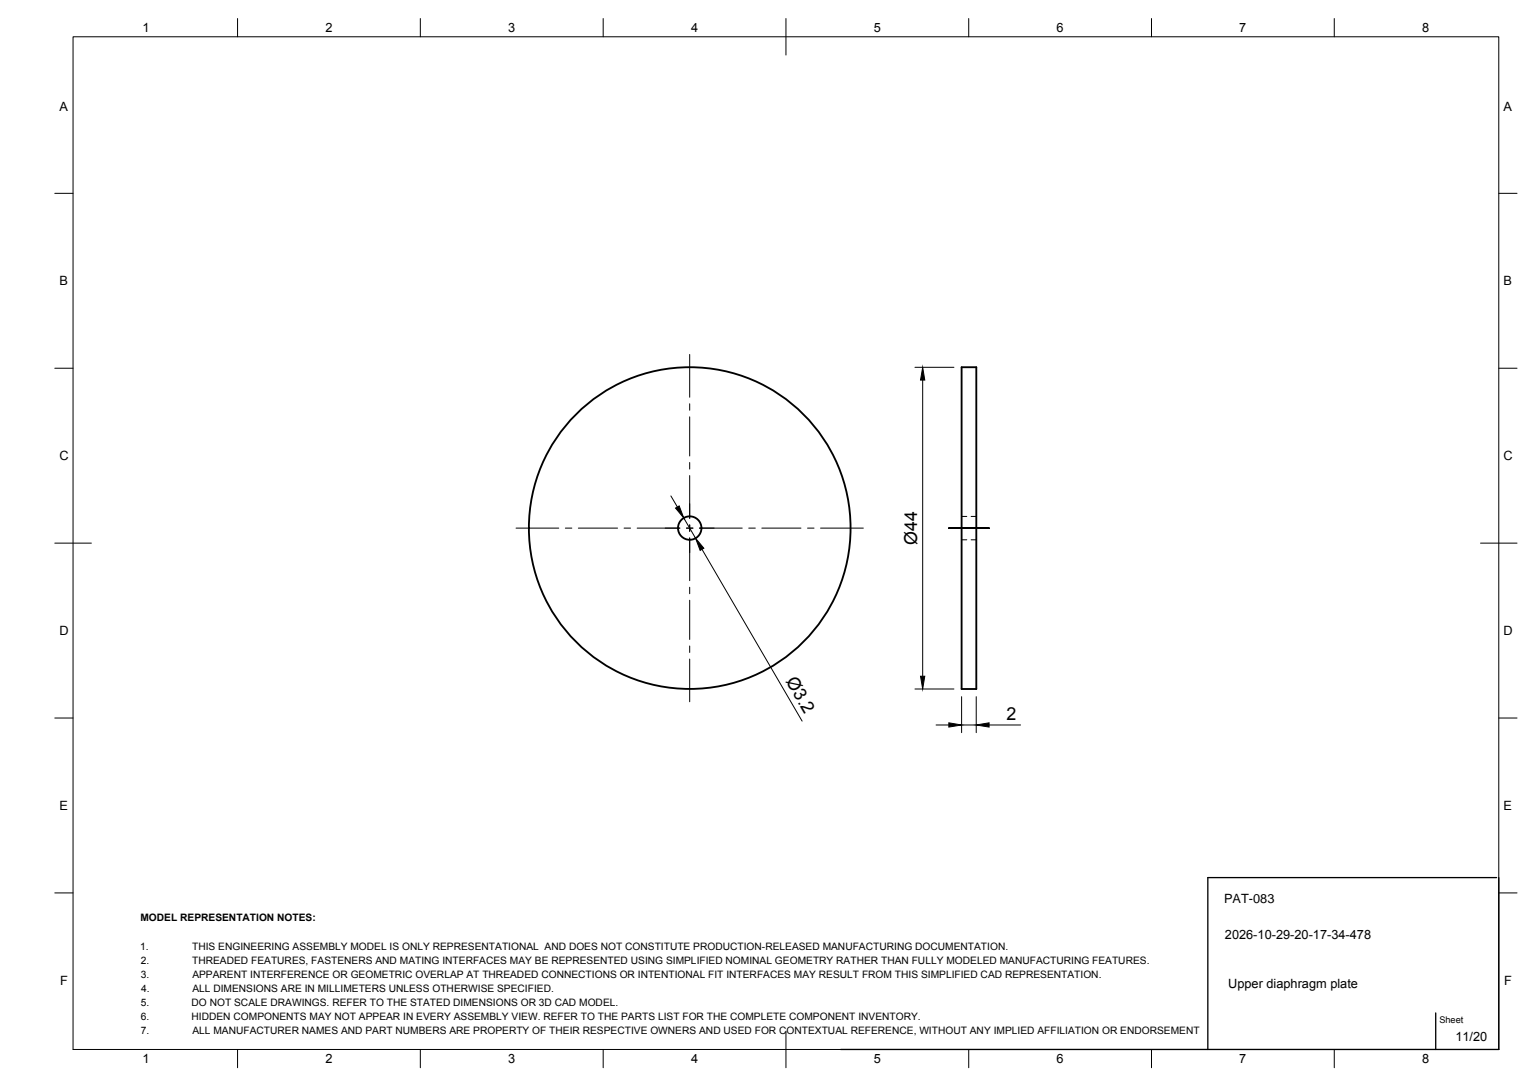
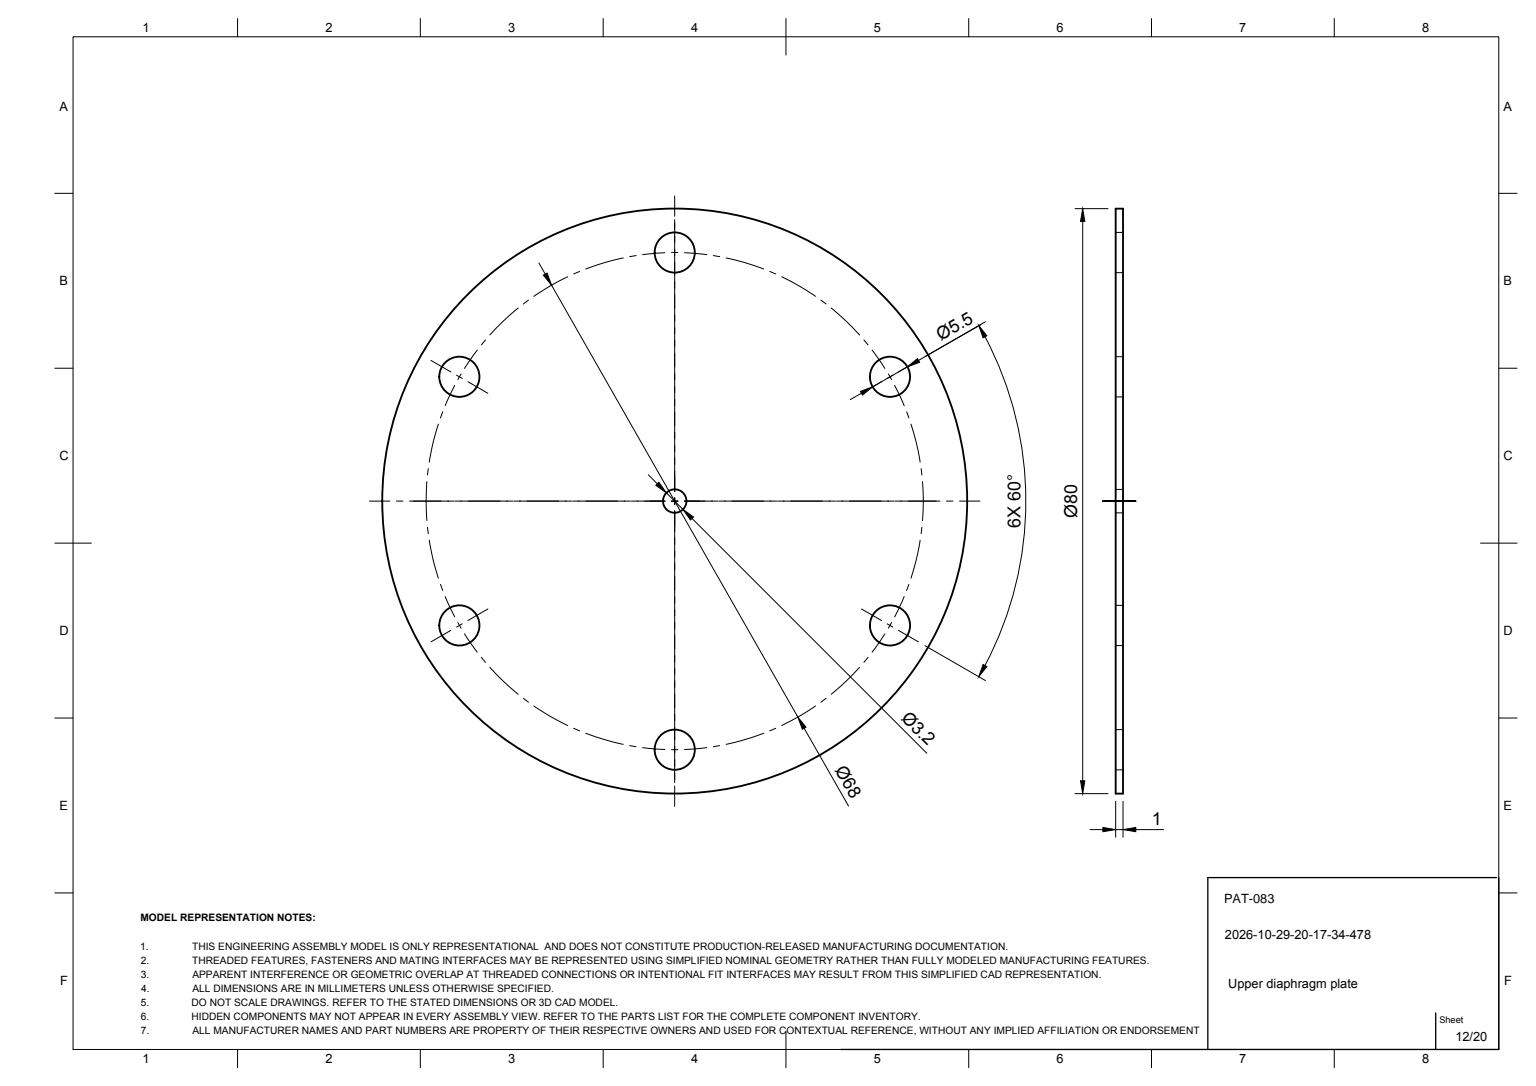
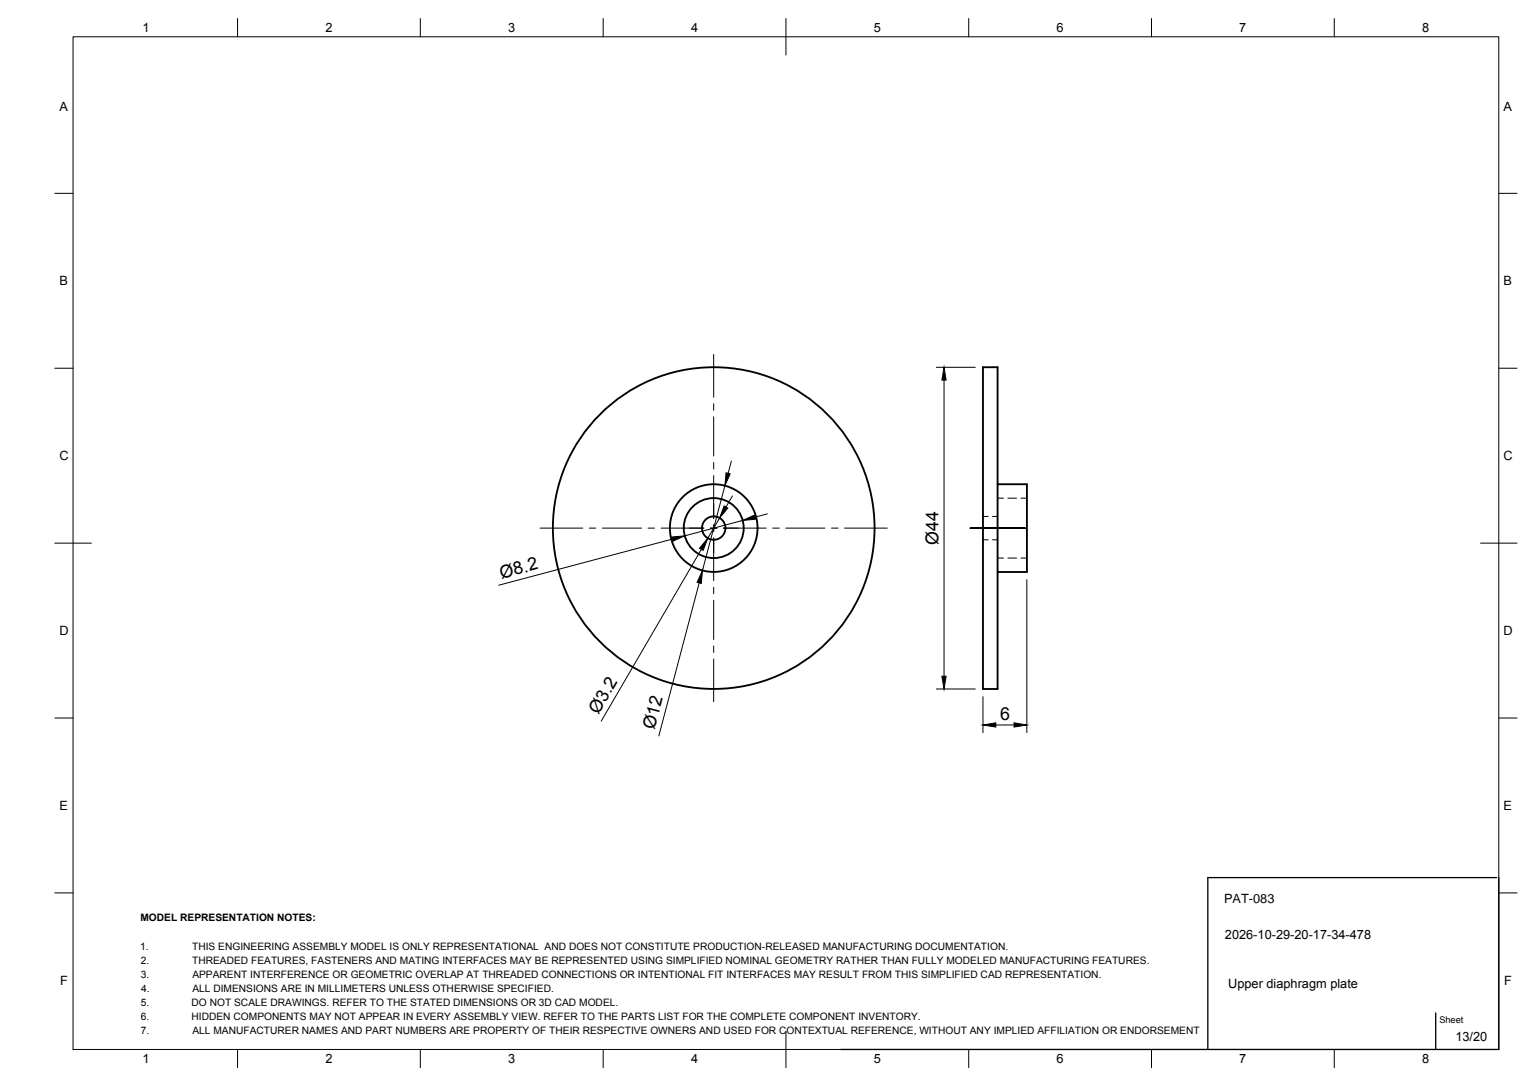
ISO-10303-21;
HEADER;
/* Generated by software containing ST-Developer
 * from STEP Tools, Inc. (www.steptools.com) 
 */

FILE_DESCRIPTION(
/* description */ ('PAT-083'),
/* implementation_level */ '2;1');

FILE_NAME(
/* name */ 'Upper diaphragm plate.step',
/* time_stamp */ '2026-10-29T20:18:00-07:00',
/* author */ (''),
/* organization */ (''),
/* preprocessor_version */ 'ST-DEVELOPER v20.2',
/* originating_system */ 'Autodesk Translation Framework v15.17.0.0',
/* authorisation */ '');

FILE_SCHEMA (('AUTOMOTIVE_DESIGN { 1 0 10303 214 3 1 1 }'));
ENDSEC;

DATA;
#10=MECHANICAL_DESIGN_GEOMETRIC_PRESENTATION_REPRESENTATION('',(#239),#8428);
#191=SHAPE_REPRESENTATION_RELATIONSHIP('SRR','None',#8525,#215);
#215=ADVANCED_BREP_SHAPE_REPRESENTATION('',(#263),#8414);
#239=STYLED_ITEM('',(#8698),#263);
#263=MANIFOLD_SOLID_BREP('Body1',#3685);
#320=FACE_BOUND('',#869,.T.);
#321=FACE_BOUND('',#871,.T.);
#322=FACE_BOUND('',#875,.T.);
#323=FACE_BOUND('',#877,.T.);
#407=PLANE('',#4156);
#408=PLANE('',#4157);
#409=PLANE('',#4164);
#410=PLANE('',#4165);
#588=FACE_OUTER_BOUND('',#866,.T.);
#589=FACE_OUTER_BOUND('',#867,.T.);
#590=FACE_OUTER_BOUND('',#868,.T.);
#591=FACE_OUTER_BOUND('',#870,.T.);
#592=FACE_OUTER_BOUND('',#872,.T.);
#593=FACE_OUTER_BOUND('',#873,.T.);
#594=FACE_OUTER_BOUND('',#874,.T.);
#595=FACE_OUTER_BOUND('',#876,.T.);
#866=EDGE_LOOP('',(#2804,#2805,#2806,#2807));
#867=EDGE_LOOP('',(#2808,#2809,#2810,#2811));
#868=EDGE_LOOP('',(#2812));
#869=EDGE_LOOP('',(#2813));
#870=EDGE_LOOP('',(#2814));
#871=EDGE_LOOP('',(#2815));
#872=EDGE_LOOP('',(#2816,#2817,#2818,#2819));
#873=EDGE_LOOP('',(#2820,#2821,#2822,#2823));
#874=EDGE_LOOP('',(#2824));
#875=EDGE_LOOP('',(#2825));
#876=EDGE_LOOP('',(#2826));
#877=EDGE_LOOP('',(#2827));
#1125=LINE('',#6881,#1369);
#1126=LINE('',#6887,#1370);
#1127=LINE('',#6897,#1371);
#1128=LINE('',#6901,#1372);
#1369=VECTOR('',#4891,0.41);
#1370=VECTOR('',#4898,0.6);
#1371=VECTOR('',#4911,0.16);
#1372=VECTOR('',#4916,2.2);
#1610=CIRCLE('',#4151,0.41);
#1611=CIRCLE('',#4152,0.41);
#1612=CIRCLE('',#4154,0.6);
#1613=CIRCLE('',#4155,0.6);
#1614=CIRCLE('',#4158,2.2);
#1615=CIRCLE('',#4160,0.16);
#1616=CIRCLE('',#4161,0.16);
#1617=CIRCLE('',#4163,2.2);
#1823=VERTEX_POINT('',#6878);
#1824=VERTEX_POINT('',#6880);
#1825=VERTEX_POINT('',#6884);
#1826=VERTEX_POINT('',#6886);
#1827=VERTEX_POINT('',#6891);
#1828=VERTEX_POINT('',#6894);
#1829=VERTEX_POINT('',#6896);
#1830=VERTEX_POINT('',#6900);
#2178=EDGE_CURVE('',#1823,#1823,#1610,.T.);
#2179=EDGE_CURVE('',#1823,#1824,#1125,.T.);
#2180=EDGE_CURVE('',#1824,#1824,#1611,.T.);
#2181=EDGE_CURVE('',#1825,#1825,#1612,.T.);
#2182=EDGE_CURVE('',#1825,#1826,#1126,.T.);
#2183=EDGE_CURVE('',#1826,#1826,#1613,.T.);
#2184=EDGE_CURVE('',#1827,#1827,#1614,.T.);
#2185=EDGE_CURVE('',#1828,#1828,#1615,.T.);
#2186=EDGE_CURVE('',#1828,#1829,#1127,.T.);
#2187=EDGE_CURVE('',#1829,#1829,#1616,.T.);
#2188=EDGE_CURVE('',#1827,#1830,#1128,.T.);
#2189=EDGE_CURVE('',#1830,#1830,#1617,.T.);
#2804=ORIENTED_EDGE('',*,*,#2178,.F.);
#2805=ORIENTED_EDGE('',*,*,#2179,.T.);
#2806=ORIENTED_EDGE('',*,*,#2180,.F.);
#2807=ORIENTED_EDGE('',*,*,#2179,.F.);
#2808=ORIENTED_EDGE('',*,*,#2181,.F.);
#2809=ORIENTED_EDGE('',*,*,#2182,.T.);
#2810=ORIENTED_EDGE('',*,*,#2183,.F.);
#2811=ORIENTED_EDGE('',*,*,#2182,.F.);
#2812=ORIENTED_EDGE('',*,*,#2181,.T.);
#2813=ORIENTED_EDGE('',*,*,#2178,.T.);
#2814=ORIENTED_EDGE('',*,*,#2184,.T.);
#2815=ORIENTED_EDGE('',*,*,#2183,.T.);
#2816=ORIENTED_EDGE('',*,*,#2185,.F.);
#2817=ORIENTED_EDGE('',*,*,#2186,.T.);
#2818=ORIENTED_EDGE('',*,*,#2187,.T.);
#2819=ORIENTED_EDGE('',*,*,#2186,.F.);
#2820=ORIENTED_EDGE('',*,*,#2184,.F.);
#2821=ORIENTED_EDGE('',*,*,#2188,.T.);
#2822=ORIENTED_EDGE('',*,*,#2189,.T.);
#2823=ORIENTED_EDGE('',*,*,#2188,.F.);
#2824=ORIENTED_EDGE('',*,*,#2180,.T.);
#2825=ORIENTED_EDGE('',*,*,#2185,.T.);
#2826=ORIENTED_EDGE('',*,*,#2189,.F.);
#2827=ORIENTED_EDGE('',*,*,#2187,.F.);
#3405=CYLINDRICAL_SURFACE('',#4150,0.41);
#3406=CYLINDRICAL_SURFACE('',#4153,0.6);
#3407=CYLINDRICAL_SURFACE('',#4159,0.16);
#3408=CYLINDRICAL_SURFACE('',#4162,2.2);
#3535=ADVANCED_FACE('',(#588),#3405,.F.);
#3536=ADVANCED_FACE('',(#589),#3406,.T.);
#3537=ADVANCED_FACE('',(#590,#320),#407,.T.);
#3538=ADVANCED_FACE('',(#591,#321),#408,.T.);
#3539=ADVANCED_FACE('',(#592),#3407,.F.);
#3540=ADVANCED_FACE('',(#593),#3408,.T.);
#3541=ADVANCED_FACE('',(#594,#322),#409,.T.);
#3542=ADVANCED_FACE('',(#595,#323),#410,.F.);
#3685=CLOSED_SHELL('',(#3535,#3536,#3537,#3538,#3539,#3540,#3541,#3542));
#4149=AXIS2_PLACEMENT_3D('',#6876,#4885,#4886);
#4150=AXIS2_PLACEMENT_3D('',#6877,#4887,#4888);
#4151=AXIS2_PLACEMENT_3D('',#6879,#4889,#4890);
#4152=AXIS2_PLACEMENT_3D('',#6882,#4892,#4893);
#4153=AXIS2_PLACEMENT_3D('',#6883,#4894,#4895);
#4154=AXIS2_PLACEMENT_3D('',#6885,#4896,#4897);
#4155=AXIS2_PLACEMENT_3D('',#6888,#4899,#4900);
#4156=AXIS2_PLACEMENT_3D('',#6889,#4901,#4902);
#4157=AXIS2_PLACEMENT_3D('',#6890,#4903,#4904);
#4158=AXIS2_PLACEMENT_3D('',#6892,#4905,#4906);
#4159=AXIS2_PLACEMENT_3D('',#6893,#4907,#4908);
#4160=AXIS2_PLACEMENT_3D('',#6895,#4909,#4910);
#4161=AXIS2_PLACEMENT_3D('',#6898,#4912,#4913);
#4162=AXIS2_PLACEMENT_3D('',#6899,#4914,#4915);
#4163=AXIS2_PLACEMENT_3D('',#6902,#4917,#4918);
#4164=AXIS2_PLACEMENT_3D('',#6903,#4919,#4920);
#4165=AXIS2_PLACEMENT_3D('',#6904,#4921,#4922);
#4885=DIRECTION('axis',(0.,0.,1.));
#4886=DIRECTION('refdir',(1.,0.,0.));
#4887=DIRECTION('center_axis',(0.,0.,1.));
#4888=DIRECTION('ref_axis',(1.,0.,0.));
#4889=DIRECTION('center_axis',(0.,0.,-1.));
#4890=DIRECTION('ref_axis',(1.,0.,0.));
#4891=DIRECTION('',(0.,0.,-1.));
#4892=DIRECTION('center_axis',(0.,0.,1.));
#4893=DIRECTION('ref_axis',(1.,0.,0.));
#4894=DIRECTION('center_axis',(0.,0.,1.));
#4895=DIRECTION('ref_axis',(1.,0.,0.));
#4896=DIRECTION('center_axis',(0.,0.,1.));
#4897=DIRECTION('ref_axis',(1.,0.,0.));
#4898=DIRECTION('',(0.,0.,-1.));
#4899=DIRECTION('center_axis',(0.,0.,-1.));
#4900=DIRECTION('ref_axis',(1.,0.,0.));
#4901=DIRECTION('center_axis',(0.,0.,1.));
#4902=DIRECTION('ref_axis',(1.,0.,0.));
#4903=DIRECTION('center_axis',(0.,0.,1.));
#4904=DIRECTION('ref_axis',(1.,0.,0.));
#4905=DIRECTION('center_axis',(0.,0.,1.));
#4906=DIRECTION('ref_axis',(1.,0.,0.));
#4907=DIRECTION('center_axis',(0.,0.,1.));
#4908=DIRECTION('ref_axis',(1.,0.,0.));
#4909=DIRECTION('center_axis',(0.,0.,-1.));
#4910=DIRECTION('ref_axis',(1.,0.,0.));
#4911=DIRECTION('',(0.,0.,-1.));
#4912=DIRECTION('center_axis',(0.,0.,-1.));
#4913=DIRECTION('ref_axis',(1.,0.,0.));
#4914=DIRECTION('center_axis',(0.,0.,1.));
#4915=DIRECTION('ref_axis',(1.,0.,0.));
#4916=DIRECTION('',(0.,0.,-1.));
#4917=DIRECTION('center_axis',(0.,0.,1.));
#4918=DIRECTION('ref_axis',(1.,0.,0.));
#4919=DIRECTION('center_axis',(0.,0.,1.));
#4920=DIRECTION('ref_axis',(1.,0.,0.));
#4921=DIRECTION('center_axis',(0.,0.,1.));
#4922=DIRECTION('ref_axis',(1.,0.,0.));
#6876=CARTESIAN_POINT('',(0.,0.,0.));
#6877=CARTESIAN_POINT('Origin',(0.,0.,5.3));
#6878=CARTESIAN_POINT('',(-0.41,-5.02105187650415E-17,5.7));
#6879=CARTESIAN_POINT('Origin',(0.,0.,5.7));
#6880=CARTESIAN_POINT('',(-0.41,-5.02105187650415E-17,5.3));
#6881=CARTESIAN_POINT('',(-0.41,-5.02105187650415E-17,5.3));
#6882=CARTESIAN_POINT('Origin',(0.,0.,5.3));
#6883=CARTESIAN_POINT('Origin',(0.,0.,5.3));
#6884=CARTESIAN_POINT('',(-0.6,-7.34788079488412E-17,5.7));
#6885=CARTESIAN_POINT('Origin',(0.,0.,5.7));
#6886=CARTESIAN_POINT('',(-0.6,-7.34788079488412E-17,5.3));
#6887=CARTESIAN_POINT('',(-0.6,-7.34788079488412E-17,5.3));
#6888=CARTESIAN_POINT('Origin',(0.,0.,5.3));
#6889=CARTESIAN_POINT('Origin',(0.,0.,5.7));
#6890=CARTESIAN_POINT('Origin',(0.,0.,5.3));
#6891=CARTESIAN_POINT('',(-2.2,-2.69422295812418E-16,5.3));
#6892=CARTESIAN_POINT('Origin',(0.,0.,5.3));
#6893=CARTESIAN_POINT('Origin',(0.,0.,5.1));
#6894=CARTESIAN_POINT('',(-0.16,-1.95943487863577E-17,5.3));
#6895=CARTESIAN_POINT('Origin',(0.,0.,5.3));
#6896=CARTESIAN_POINT('',(-0.16,-1.95943487863577E-17,5.1));
#6897=CARTESIAN_POINT('',(-0.16,-1.95943487863577E-17,5.1));
#6898=CARTESIAN_POINT('Origin',(0.,0.,5.1));
#6899=CARTESIAN_POINT('Origin',(0.,0.,5.1));
#6900=CARTESIAN_POINT('',(-2.2,-2.69422295812418E-16,5.1));
#6901=CARTESIAN_POINT('',(-2.2,-2.69422295812418E-16,5.1));
#6902=CARTESIAN_POINT('Origin',(0.,0.,5.1));
#6903=CARTESIAN_POINT('Origin',(0.,0.,5.3));
#6904=CARTESIAN_POINT('Origin',(0.,0.,5.1));
#8388=UNCERTAINTY_MEASURE_WITH_UNIT(LENGTH_MEASURE(0.001),#8429,
'DISTANCE_ACCURACY_VALUE',
'Maximum model space distance between geometric entities at asserted c
onnectivities');
#8402=UNCERTAINTY_MEASURE_WITH_UNIT(LENGTH_MEASURE(0.001),#8429,
'DISTANCE_ACCURACY_VALUE',
'Maximum model space distance between geometric entities at asserted c
onnectivities');
#8414=(
GEOMETRIC_REPRESENTATION_CONTEXT(3)
GLOBAL_UNCERTAINTY_ASSIGNED_CONTEXT((#8388))
GLOBAL_UNIT_ASSIGNED_CONTEXT((#8429,#8431,#8432))
REPRESENTATION_CONTEXT('','3D')
);
#8428=(
GEOMETRIC_REPRESENTATION_CONTEXT(3)
GLOBAL_UNCERTAINTY_ASSIGNED_CONTEXT((#8402))
GLOBAL_UNIT_ASSIGNED_CONTEXT((#8429,#8431,#8432))
REPRESENTATION_CONTEXT('','3D')
);
#8429=(
LENGTH_UNIT()
NAMED_UNIT(*)
SI_UNIT(.CENTI.,.METRE.)
);
#8431=(
NAMED_UNIT(*)
PLANE_ANGLE_UNIT()
SI_UNIT($,.RADIAN.)
);
#8432=(
NAMED_UNIT(*)
SI_UNIT($,.STERADIAN.)
SOLID_ANGLE_UNIT()
);
#8444=SHAPE_DEFINITION_REPRESENTATION(#8469,#8525);
#8469=PRODUCT_DEFINITION_SHAPE('',$,#8551);
#8525=SHAPE_REPRESENTATION('',(#4149),#8414);
#8539=PRODUCT_DEFINITION_CONTEXT('part definition',#8616,'design');
#8551=PRODUCT_DEFINITION('Upper diaphragm plate',
'Upper diaphragm plate',#8576,#8539);
#8576=PRODUCT_DEFINITION_FORMATION('',$,#8629);
#8616=APPLICATION_CONTEXT(
'Core Data for Automotive Mechanical Design Process');
#8617=PRODUCT_CONTEXT('part definition',#8616,'mechanical');
#8629=PRODUCT('Upper diaphragm plate','Upper diaphragm plate',
'Upper diaphragm plate',(#8617));
#8692=COLOUR_RGB('Sky Blue',0.24,0.69,0.87);
#8693=FILL_AREA_STYLE_COLOUR('',#8692);
#8694=FILL_AREA_STYLE('',(#8693));
#8695=SURFACE_STYLE_FILL_AREA(#8694);
#8696=SURFACE_SIDE_STYLE('',(#8695));
#8697=SURFACE_STYLE_USAGE(.BOTH.,#8696);
#8698=PRESENTATION_STYLE_ASSIGNMENT((#8697));
ENDSEC;
END-ISO-10303-21;
